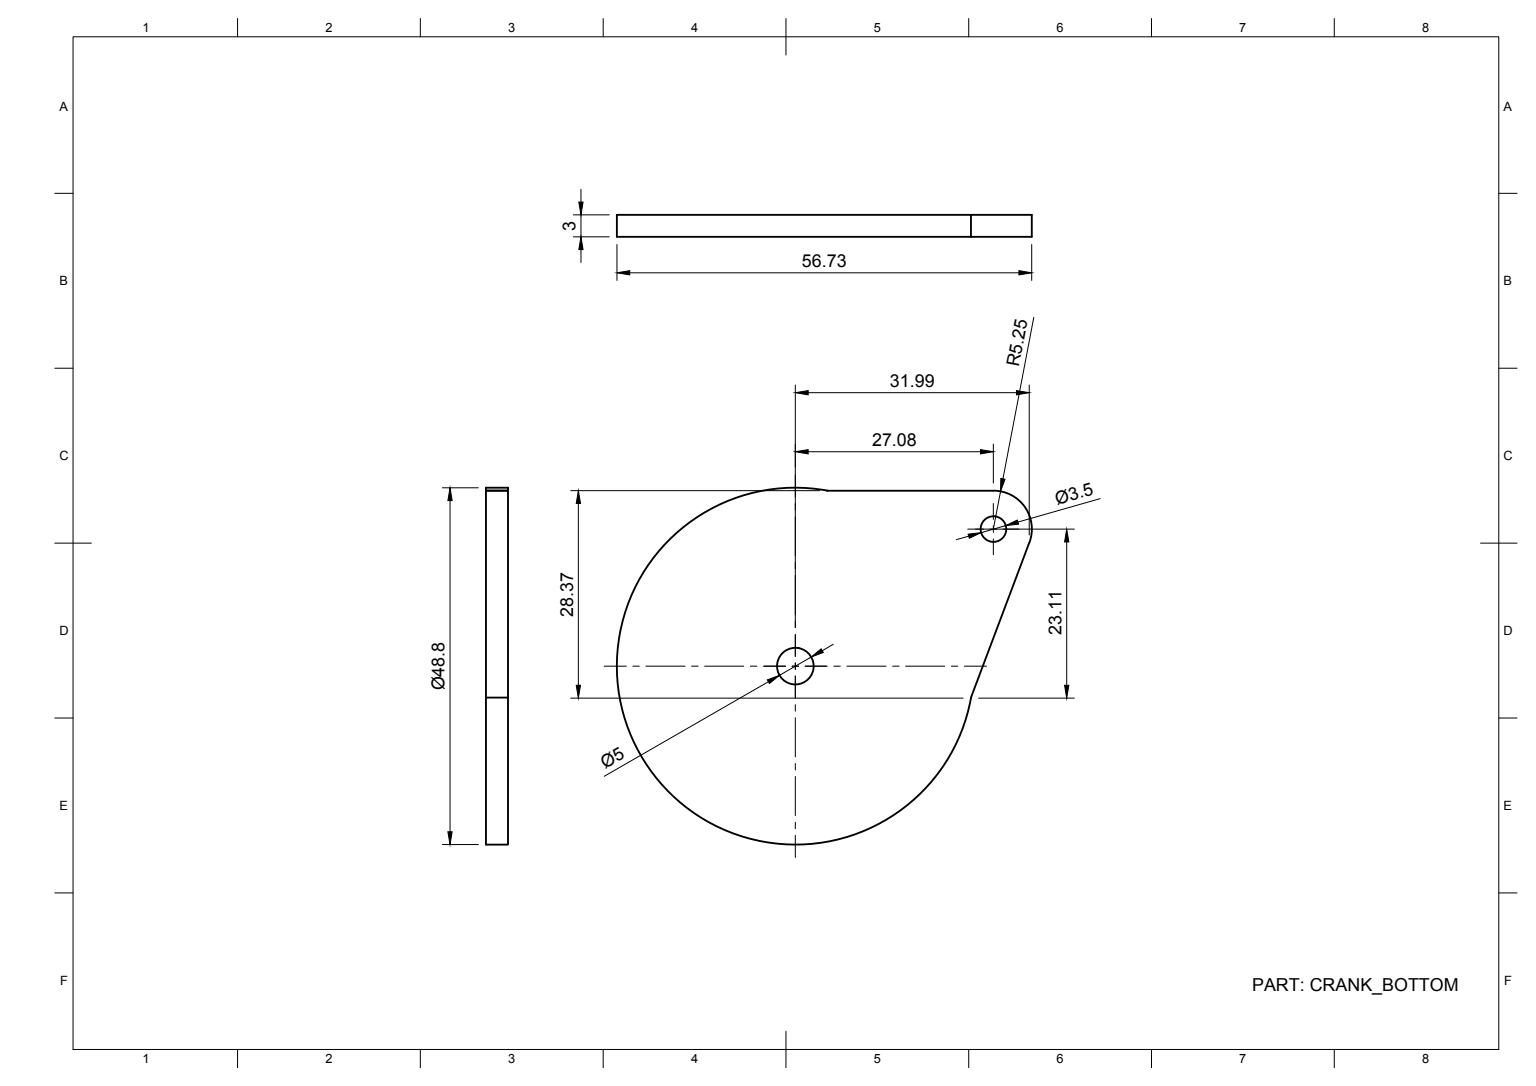
ISO-10303-21;
HEADER;
/* Generated by software containing ST-Developer
 * from STEP Tools, Inc. (www.steptools.com) 
 */

FILE_DESCRIPTION(
/* description */ (''),
/* implementation_level */ '2;1');

FILE_NAME(
/* name */ 'Crank_Bottom.step',
/* time_stamp */ '2026-09-20T21:52:48+06:00',
/* author */ (''),
/* organization */ (''),
/* preprocessor_version */ 'ST-DEVELOPER v20.2',
/* originating_system */ 'Autodesk Translation Framework v15.15.0.0',
/* authorisation */ '');

FILE_SCHEMA (('AUTOMOTIVE_DESIGN { 1 0 10303 214 3 1 1 }'));
ENDSEC;

DATA;
#10=MECHANICAL_DESIGN_GEOMETRIC_PRESENTATION_REPRESENTATION('',(#63),#2203);
#47=SHAPE_REPRESENTATION_RELATIONSHIP('SRR','None',#2239,#55);
#55=ADVANCED_BREP_SHAPE_REPRESENTATION('',(#71),#2199);
#63=STYLED_ITEM('',(#2285),#71);
#71=MANIFOLD_SOLID_BREP('Crank_Bottom',#1230);
#81=FACE_BOUND('',#280,.T.);
#82=FACE_BOUND('',#281,.T.);
#83=FACE_BOUND('',#288,.T.);
#84=FACE_BOUND('',#289,.T.);
#115=CIRCLE('',#1399,5.25);
#116=CIRCLE('',#1400,24.399223777829);
#117=CIRCLE('',#1401,2.5);
#118=CIRCLE('',#1402,1.75);
#119=CIRCLE('',#1405,5.25);
#120=CIRCLE('',#1407,1.75);
#121=CIRCLE('',#1410,2.5);
#122=CIRCLE('',#1412,24.399223777829);
#150=CYLINDRICAL_SURFACE('',#1404,5.25);
#151=CYLINDRICAL_SURFACE('',#1406,1.75);
#152=CYLINDRICAL_SURFACE('',#1409,2.5);
#153=CYLINDRICAL_SURFACE('',#1413,24.399223777829);
#202=FACE_OUTER_BOUND('',#277,.T.);
#203=FACE_OUTER_BOUND('',#278,.T.);
#204=FACE_OUTER_BOUND('',#279,.T.);
#205=FACE_OUTER_BOUND('',#282,.T.);
#206=FACE_OUTER_BOUND('',#283,.T.);
#207=FACE_OUTER_BOUND('',#284,.T.);
#208=FACE_OUTER_BOUND('',#285,.T.);
#209=FACE_OUTER_BOUND('',#286,.T.);
#210=FACE_OUTER_BOUND('',#287,.T.);
#211=FACE_OUTER_BOUND('',#290,.T.);
#277=EDGE_LOOP('',(#994,#995,#996,#997));
#278=EDGE_LOOP('',(#998,#999,#1000,#1001));
#279=EDGE_LOOP('',(#1002,#1003,#1004,#1005,#1006,#1007));
#280=EDGE_LOOP('',(#1008));
#281=EDGE_LOOP('',(#1009));
#282=EDGE_LOOP('',(#1010,#1011,#1012,#1013));
#283=EDGE_LOOP('',(#1014,#1015,#1016,#1017));
#284=EDGE_LOOP('',(#1018,#1019,#1020,#1021));
#285=EDGE_LOOP('',(#1022,#1023,#1024,#1025));
#286=EDGE_LOOP('',(#1026,#1027,#1028,#1029));
#287=EDGE_LOOP('',(#1030,#1031,#1032,#1033,#1034,#1035));
#288=EDGE_LOOP('',(#1036));
#289=EDGE_LOOP('',(#1037));
#290=EDGE_LOOP('',(#1038,#1039,#1040,#1041));
#386=LINE('',#2050,#496);
#387=LINE('',#2052,#497);
#388=LINE('',#2054,#498);
#389=LINE('',#2055,#499);
#390=LINE('',#2059,#500);
#391=LINE('',#2061,#501);
#392=LINE('',#2063,#502);
#393=LINE('',#2064,#503);
#394=LINE('',#2067,#504);
#395=LINE('',#2070,#505);
#396=LINE('',#2078,#506);
#397=LINE('',#2079,#507);
#398=LINE('',#2084,#508);
#399=LINE('',#2088,#509);
#400=LINE('',#2089,#510);
#401=LINE('',#2092,#511);
#496=VECTOR('',#1678,10.);
#497=VECTOR('',#1679,10.);
#498=VECTOR('',#1680,10.);
#499=VECTOR('',#1681,10.);
#500=VECTOR('',#1684,10.);
#501=VECTOR('',#1685,10.);
#502=VECTOR('',#1686,10.);
#503=VECTOR('',#1687,10.);
#504=VECTOR('',#1690,10.);
#505=VECTOR('',#1693,10.);
#506=VECTOR('',#1702,10.);
#507=VECTOR('',#1703,10.);
#508=VECTOR('',#1710,1.75);
#509=VECTOR('',#1715,10.);
#510=VECTOR('',#1716,10.);
#511=VECTOR('',#1719,2.5);
#599=VERTEX_POINT('',#2048);
#600=VERTEX_POINT('',#2049);
#601=VERTEX_POINT('',#2051);
#602=VERTEX_POINT('',#2053);
#603=VERTEX_POINT('',#2057);
#604=VERTEX_POINT('',#2058);
#605=VERTEX_POINT('',#2060);
#606=VERTEX_POINT('',#2062);
#607=VERTEX_POINT('',#2066);
#608=VERTEX_POINT('',#2069);
#609=VERTEX_POINT('',#2072);
#610=VERTEX_POINT('',#2074);
#611=VERTEX_POINT('',#2077);
#612=VERTEX_POINT('',#2083);
#613=VERTEX_POINT('',#2087);
#614=VERTEX_POINT('',#2091);
#737=EDGE_CURVE('',#599,#600,#386,.T.);
#738=EDGE_CURVE('',#600,#601,#387,.T.);
#739=EDGE_CURVE('',#602,#601,#388,.T.);
#740=EDGE_CURVE('',#599,#602,#389,.T.);
#741=EDGE_CURVE('',#603,#604,#390,.T.);
#742=EDGE_CURVE('',#604,#605,#391,.T.);
#743=EDGE_CURVE('',#606,#605,#392,.T.);
#744=EDGE_CURVE('',#603,#606,#393,.T.);
#745=EDGE_CURVE('',#605,#607,#394,.T.);
#746=EDGE_CURVE('',#607,#602,#115,.T.);
#747=EDGE_CURVE('',#601,#608,#395,.T.);
#748=EDGE_CURVE('',#606,#608,#116,.T.);
#749=EDGE_CURVE('',#609,#609,#117,.T.);
#750=EDGE_CURVE('',#610,#610,#118,.T.);
#751=EDGE_CURVE('',#604,#611,#396,.T.);
#752=EDGE_CURVE('',#611,#607,#397,.T.);
#753=EDGE_CURVE('',#611,#599,#119,.T.);
#754=EDGE_CURVE('',#610,#612,#398,.T.);
#755=EDGE_CURVE('',#612,#612,#120,.T.);
#756=EDGE_CURVE('',#600,#613,#399,.T.);
#757=EDGE_CURVE('',#608,#613,#400,.T.);
#758=EDGE_CURVE('',#609,#614,#401,.T.);
#759=EDGE_CURVE('',#614,#614,#121,.T.);
#760=EDGE_CURVE('',#613,#603,#122,.T.);
#994=ORIENTED_EDGE('',*,*,#737,.T.);
#995=ORIENTED_EDGE('',*,*,#738,.T.);
#996=ORIENTED_EDGE('',*,*,#739,.F.);
#997=ORIENTED_EDGE('',*,*,#740,.F.);
#998=ORIENTED_EDGE('',*,*,#741,.T.);
#999=ORIENTED_EDGE('',*,*,#742,.T.);
#1000=ORIENTED_EDGE('',*,*,#743,.F.);
#1001=ORIENTED_EDGE('',*,*,#744,.F.);
#1002=ORIENTED_EDGE('',*,*,#743,.T.);
#1003=ORIENTED_EDGE('',*,*,#745,.T.);
#1004=ORIENTED_EDGE('',*,*,#746,.T.);
#1005=ORIENTED_EDGE('',*,*,#739,.T.);
#1006=ORIENTED_EDGE('',*,*,#747,.T.);
#1007=ORIENTED_EDGE('',*,*,#748,.F.);
#1008=ORIENTED_EDGE('',*,*,#749,.T.);
#1009=ORIENTED_EDGE('',*,*,#750,.T.);
#1010=ORIENTED_EDGE('',*,*,#751,.T.);
#1011=ORIENTED_EDGE('',*,*,#752,.T.);
#1012=ORIENTED_EDGE('',*,*,#745,.F.);
#1013=ORIENTED_EDGE('',*,*,#742,.F.);
#1014=ORIENTED_EDGE('',*,*,#740,.T.);
#1015=ORIENTED_EDGE('',*,*,#746,.F.);
#1016=ORIENTED_EDGE('',*,*,#752,.F.);
#1017=ORIENTED_EDGE('',*,*,#753,.T.);
#1018=ORIENTED_EDGE('',*,*,#750,.F.);
#1019=ORIENTED_EDGE('',*,*,#754,.T.);
#1020=ORIENTED_EDGE('',*,*,#755,.F.);
#1021=ORIENTED_EDGE('',*,*,#754,.F.);
#1022=ORIENTED_EDGE('',*,*,#756,.T.);
#1023=ORIENTED_EDGE('',*,*,#757,.F.);
#1024=ORIENTED_EDGE('',*,*,#747,.F.);
#1025=ORIENTED_EDGE('',*,*,#738,.F.);
#1026=ORIENTED_EDGE('',*,*,#749,.F.);
#1027=ORIENTED_EDGE('',*,*,#758,.T.);
#1028=ORIENTED_EDGE('',*,*,#759,.T.);
#1029=ORIENTED_EDGE('',*,*,#758,.F.);
#1030=ORIENTED_EDGE('',*,*,#737,.F.);
#1031=ORIENTED_EDGE('',*,*,#753,.F.);
#1032=ORIENTED_EDGE('',*,*,#751,.F.);
#1033=ORIENTED_EDGE('',*,*,#741,.F.);
#1034=ORIENTED_EDGE('',*,*,#760,.F.);
#1035=ORIENTED_EDGE('',*,*,#756,.F.);
#1036=ORIENTED_EDGE('',*,*,#759,.F.);
#1037=ORIENTED_EDGE('',*,*,#755,.T.);
#1038=ORIENTED_EDGE('',*,*,#760,.T.);
#1039=ORIENTED_EDGE('',*,*,#744,.T.);
#1040=ORIENTED_EDGE('',*,*,#748,.T.);
#1041=ORIENTED_EDGE('',*,*,#757,.T.);
#1140=PLANE('',#1396);
#1141=PLANE('',#1397);
#1142=PLANE('',#1398);
#1143=PLANE('',#1403);
#1144=PLANE('',#1408);
#1145=PLANE('',#1411);
#1198=ADVANCED_FACE('',(#202),#1140,.T.);
#1199=ADVANCED_FACE('',(#203),#1141,.F.);
#1200=ADVANCED_FACE('',(#204,#81,#82),#1142,.T.);
#1201=ADVANCED_FACE('',(#205),#1143,.T.);
#1202=ADVANCED_FACE('',(#206),#150,.T.);
#1203=ADVANCED_FACE('',(#207),#151,.F.);
#1204=ADVANCED_FACE('',(#208),#1144,.T.);
#1205=ADVANCED_FACE('',(#209),#152,.F.);
#1206=ADVANCED_FACE('',(#210,#83,#84),#1145,.F.);
#1207=ADVANCED_FACE('',(#211),#153,.T.);
#1230=CLOSED_SHELL('',(#1198,#1199,#1200,#1201,#1202,#1203,#1204,#1205,
#1206,#1207));
#1395=AXIS2_PLACEMENT_3D('',#2046,#1674,#1675);
#1396=AXIS2_PLACEMENT_3D('',#2047,#1676,#1677);
#1397=AXIS2_PLACEMENT_3D('',#2056,#1682,#1683);
#1398=AXIS2_PLACEMENT_3D('',#2065,#1688,#1689);
#1399=AXIS2_PLACEMENT_3D('',#2068,#1691,#1692);
#1400=AXIS2_PLACEMENT_3D('',#2071,#1694,#1695);
#1401=AXIS2_PLACEMENT_3D('',#2073,#1696,#1697);
#1402=AXIS2_PLACEMENT_3D('',#2075,#1698,#1699);
#1403=AXIS2_PLACEMENT_3D('',#2076,#1700,#1701);
#1404=AXIS2_PLACEMENT_3D('',#2080,#1704,#1705);
#1405=AXIS2_PLACEMENT_3D('',#2081,#1706,#1707);
#1406=AXIS2_PLACEMENT_3D('',#2082,#1708,#1709);
#1407=AXIS2_PLACEMENT_3D('',#2085,#1711,#1712);
#1408=AXIS2_PLACEMENT_3D('',#2086,#1713,#1714);
#1409=AXIS2_PLACEMENT_3D('',#2090,#1717,#1718);
#1410=AXIS2_PLACEMENT_3D('',#2093,#1720,#1721);
#1411=AXIS2_PLACEMENT_3D('',#2094,#1722,#1723);
#1412=AXIS2_PLACEMENT_3D('',#2095,#1724,#1725);
#1413=AXIS2_PLACEMENT_3D('',#2096,#1726,#1727);
#1674=DIRECTION('axis',(0.,0.,1.));
#1675=DIRECTION('refdir',(1.,0.,0.));
#1676=DIRECTION('center_axis',(0.983844577872192,0.,-0.179024709443944));
#1677=DIRECTION('ref_axis',(-0.179024709443944,0.,-0.983844577872192));
#1678=DIRECTION('',(-0.179024709443944,0.,-0.983844577872192));
#1679=DIRECTION('',(0.,1.,0.));
#1680=DIRECTION('',(-0.179024709443944,0.,-0.983844577872192));
#1681=DIRECTION('',(0.,1.,0.));
#1682=DIRECTION('center_axis',(-0.00140955899906737,0.,-0.999999006571221));
#1683=DIRECTION('ref_axis',(-0.999999006571221,0.,0.00140955899906737));
#1684=DIRECTION('',(0.999999006571221,0.,-0.00140955899906737));
#1685=DIRECTION('',(0.,1.,0.));
#1686=DIRECTION('',(0.999999006571221,0.,-0.00140955899906737));
#1687=DIRECTION('',(0.,1.,0.));
#1688=DIRECTION('center_axis',(0.,1.,0.));
#1689=DIRECTION('ref_axis',(1.,0.,0.));
#1690=DIRECTION('',(0.983844577872192,0.,0.179024709443943));
#1691=DIRECTION('center_axis',(0.,1.,0.));
#1692=DIRECTION('ref_axis',(1.,0.,0.));
#1693=DIRECTION('',(1.,0.,0.));
#1694=DIRECTION('center_axis',(0.,-1.,0.));
#1695=DIRECTION('ref_axis',(-1.,0.,0.));
#1696=DIRECTION('center_axis',(0.,-1.,0.));
#1697=DIRECTION('ref_axis',(1.,0.,0.));
#1698=DIRECTION('center_axis',(0.,-1.,0.));
#1699=DIRECTION('ref_axis',(1.,0.,0.));
#1700=DIRECTION('center_axis',(-0.179024709443943,0.,0.983844577872192));
#1701=DIRECTION('ref_axis',(0.983844577872192,0.,0.179024709443943));
#1702=DIRECTION('',(0.983844577872192,0.,0.179024709443943));
#1703=DIRECTION('',(0.,1.,0.));
#1704=DIRECTION('center_axis',(0.,1.,0.));
#1705=DIRECTION('ref_axis',(1.,0.,0.));
#1706=DIRECTION('center_axis',(0.,1.,0.));
#1707=DIRECTION('ref_axis',(1.,0.,0.));
#1708=DIRECTION('center_axis',(0.,-1.,0.));
#1709=DIRECTION('ref_axis',(1.,0.,0.));
#1710=DIRECTION('',(0.,-1.,0.));
#1711=DIRECTION('center_axis',(0.,1.,0.));
#1712=DIRECTION('ref_axis',(1.,0.,0.));
#1713=DIRECTION('center_axis',(0.,0.,1.));
#1714=DIRECTION('ref_axis',(1.,0.,0.));
#1715=DIRECTION('',(1.,0.,0.));
#1716=DIRECTION('',(0.,-1.,0.));
#1717=DIRECTION('center_axis',(0.,1.,0.));
#1718=DIRECTION('ref_axis',(1.,0.,0.));
#1719=DIRECTION('',(0.,-1.,0.));
#1720=DIRECTION('center_axis',(0.,-1.,0.));
#1721=DIRECTION('ref_axis',(1.,0.,0.));
#1722=DIRECTION('center_axis',(0.,1.,0.));
#1723=DIRECTION('ref_axis',(1.,0.,0.));
#1724=DIRECTION('center_axis',(0.,1.,0.));
#1725=DIRECTION('ref_axis',(-1.,0.,0.));
#1726=DIRECTION('center_axis',(0.,1.,0.));
#1727=DIRECTION('ref_axis',(-1.,0.,0.));
#2046=CARTESIAN_POINT('',(0.,0.,0.));
#2047=CARTESIAN_POINT('Origin',(27.8026817657391,0.,45.0732920359323));
#2048=CARTESIAN_POINT('',(28.4531709343409,0.,48.6481071744755));
#2049=CARTESIAN_POINT('',(24.3866105410464,0.,26.3));
#2050=CARTESIAN_POINT('',(25.9192569340967,0.,34.7227805663332));
#2051=CARTESIAN_POINT('',(24.3866105410464,3.,26.3));
#2052=CARTESIAN_POINT('',(24.3866105410464,0.,26.3));
#2053=CARTESIAN_POINT('',(28.4531709343409,3.,48.6481071744755));
#2054=CARTESIAN_POINT('',(24.3866105410464,3.,26.3));
#2055=CARTESIAN_POINT('',(28.4531709346647,0.,48.648107176255));
#2056=CARTESIAN_POINT('Origin',(0.0687842225651092,-5.,50.6991268223128));
#2057=CARTESIAN_POINT('',(0.,0.,50.699223777829));
#2058=CARTESIAN_POINT('',(0.0687842225651092,0.,50.6991268223128));
#2059=CARTESIAN_POINT('',(1.08481843563973,0.,50.6976946607217));
#2060=CARTESIAN_POINT('',(0.0687842225651103,3.,50.6991268223128));
#2061=CARTESIAN_POINT('',(0.0687842225651292,3.,50.6991268223128));
#2062=CARTESIAN_POINT('',(0.,3.,50.699223777829));
#2063=CARTESIAN_POINT('',(7.19318601548171,3.,50.6890845476763));
#2064=CARTESIAN_POINT('',(0.,3.,50.699223777829));
#2065=CARTESIAN_POINT('Origin',(14.3033855617004,3.,40.6033855617004));
#2066=CARTESIAN_POINT('',(22.3481071813648,3.,54.7531709355945));
#2067=CARTESIAN_POINT('',(4.44089209850063E-15,3.,50.6866105410464));
#2068=CARTESIAN_POINT('Origin',(23.2879869008357,3.,49.5879869008357));
#2069=CARTESIAN_POINT('',(24.399223777829,3.,26.3));
#2070=CARTESIAN_POINT('',(0.,3.,26.3));
#2071=CARTESIAN_POINT('Origin',(0.,3.,26.3));
#2072=CARTESIAN_POINT('',(-2.5,3.,26.3));
#2073=CARTESIAN_POINT('Origin',(0.,3.,26.3));
#2074=CARTESIAN_POINT('',(21.5379869008357,3.,49.5879869008357));
#2075=CARTESIAN_POINT('Origin',(23.2879869008357,3.,49.5879869008357));
#2076=CARTESIAN_POINT('Origin',(0.0687842225651098,0.,50.6991268223128));
#2077=CARTESIAN_POINT('',(22.3481071813648,0.,54.7531709355945));
#2078=CARTESIAN_POINT('',(4.44089209850063E-15,0.,50.6866105410464));
#2079=CARTESIAN_POINT('',(22.3481071813648,0.,54.7531709355945));
#2080=CARTESIAN_POINT('Origin',(23.2879869008357,0.,49.5879869008357));
#2081=CARTESIAN_POINT('Origin',(23.2879869008357,0.,49.5879869008357));
#2082=CARTESIAN_POINT('Origin',(23.2879869008357,0.,49.5879869008357));
#2083=CARTESIAN_POINT('',(21.5379869008357,0.,49.5879869008357));
#2084=CARTESIAN_POINT('',(21.5379869008357,0.,49.5879869008357));
#2085=CARTESIAN_POINT('Origin',(23.2879869008357,0.,49.5879869008357));
#2086=CARTESIAN_POINT('Origin',(24.3866105410464,0.,26.3));
#2087=CARTESIAN_POINT('',(24.399223777829,0.,26.3));
#2088=CARTESIAN_POINT('',(13.2279960512749,0.,26.3));
#2089=CARTESIAN_POINT('',(24.399223777829,3.,26.3));
#2090=CARTESIAN_POINT('Origin',(0.,0.,26.3));
#2091=CARTESIAN_POINT('',(-2.5,0.,26.3));
#2092=CARTESIAN_POINT('',(-2.5,0.,26.3));
#2093=CARTESIAN_POINT('Origin',(0.,0.,26.3));
#2094=CARTESIAN_POINT('Origin',(14.3033855617004,0.,40.6033855617004));
#2095=CARTESIAN_POINT('Origin',(0.,0.,26.3));
#2096=CARTESIAN_POINT('Origin',(0.,3.,26.3));
#2189=UNCERTAINTY_MEASURE_WITH_UNIT(LENGTH_MEASURE(0.01),#2204,
'DISTANCE_ACCURACY_VALUE',
'Maximum model space distance between geometric entities at asserted c
onnectivities');
#2193=UNCERTAINTY_MEASURE_WITH_UNIT(LENGTH_MEASURE(0.01),#2204,
'DISTANCE_ACCURACY_VALUE',
'Maximum model space distance between geometric entities at asserted c
onnectivities');
#2199=(
GEOMETRIC_REPRESENTATION_CONTEXT(3)
GLOBAL_UNCERTAINTY_ASSIGNED_CONTEXT((#2189))
GLOBAL_UNIT_ASSIGNED_CONTEXT((#2204,#2206,#2207))
REPRESENTATION_CONTEXT('','3D')
);
#2203=(
GEOMETRIC_REPRESENTATION_CONTEXT(3)
GLOBAL_UNCERTAINTY_ASSIGNED_CONTEXT((#2193))
GLOBAL_UNIT_ASSIGNED_CONTEXT((#2204,#2206,#2207))
REPRESENTATION_CONTEXT('','3D')
);
#2204=(
LENGTH_UNIT()
NAMED_UNIT(*)
SI_UNIT(.MILLI.,.METRE.)
);
#2206=(
NAMED_UNIT(*)
PLANE_ANGLE_UNIT()
SI_UNIT($,.RADIAN.)
);
#2207=(
NAMED_UNIT(*)
SI_UNIT($,.STERADIAN.)
SOLID_ANGLE_UNIT()
);
#2213=SHAPE_DEFINITION_REPRESENTATION(#2222,#2239);
#2222=PRODUCT_DEFINITION_SHAPE('',$,#2249);
#2239=SHAPE_REPRESENTATION('',(#1395),#2199);
#2243=PRODUCT_DEFINITION_CONTEXT('part definition',#2272,'design');
#2249=PRODUCT_DEFINITION('Crank_Bottom','Crank_Bottom',#2258,#2243);
#2258=PRODUCT_DEFINITION_FORMATION('',$,#2279);
#2272=APPLICATION_CONTEXT(
'Core Data for Automotive Mechanical Design Process');
#2273=PRODUCT_CONTEXT('part definition',#2272,'mechanical');
#2279=PRODUCT('Crank_Bottom','Crank_Bottom',$,(#2273));
#2285=PRESENTATION_STYLE_ASSIGNMENT((#2289));
#2289=SURFACE_STYLE_USAGE(.BOTH.,#2293);
#2293=SURFACE_SIDE_STYLE('',(#2297));
#2297=SURFACE_STYLE_FILL_AREA(#2301);
#2301=FILL_AREA_STYLE('Surface - Matte',(#2305));
#2305=FILL_AREA_STYLE_COLOUR('Surface - Matte',#2309);
#2309=COLOUR_RGB('Surface - Matte', 0.66274510, 0.83137255, 0.94901961);
ENDSEC;
END-ISO-10303-21;
